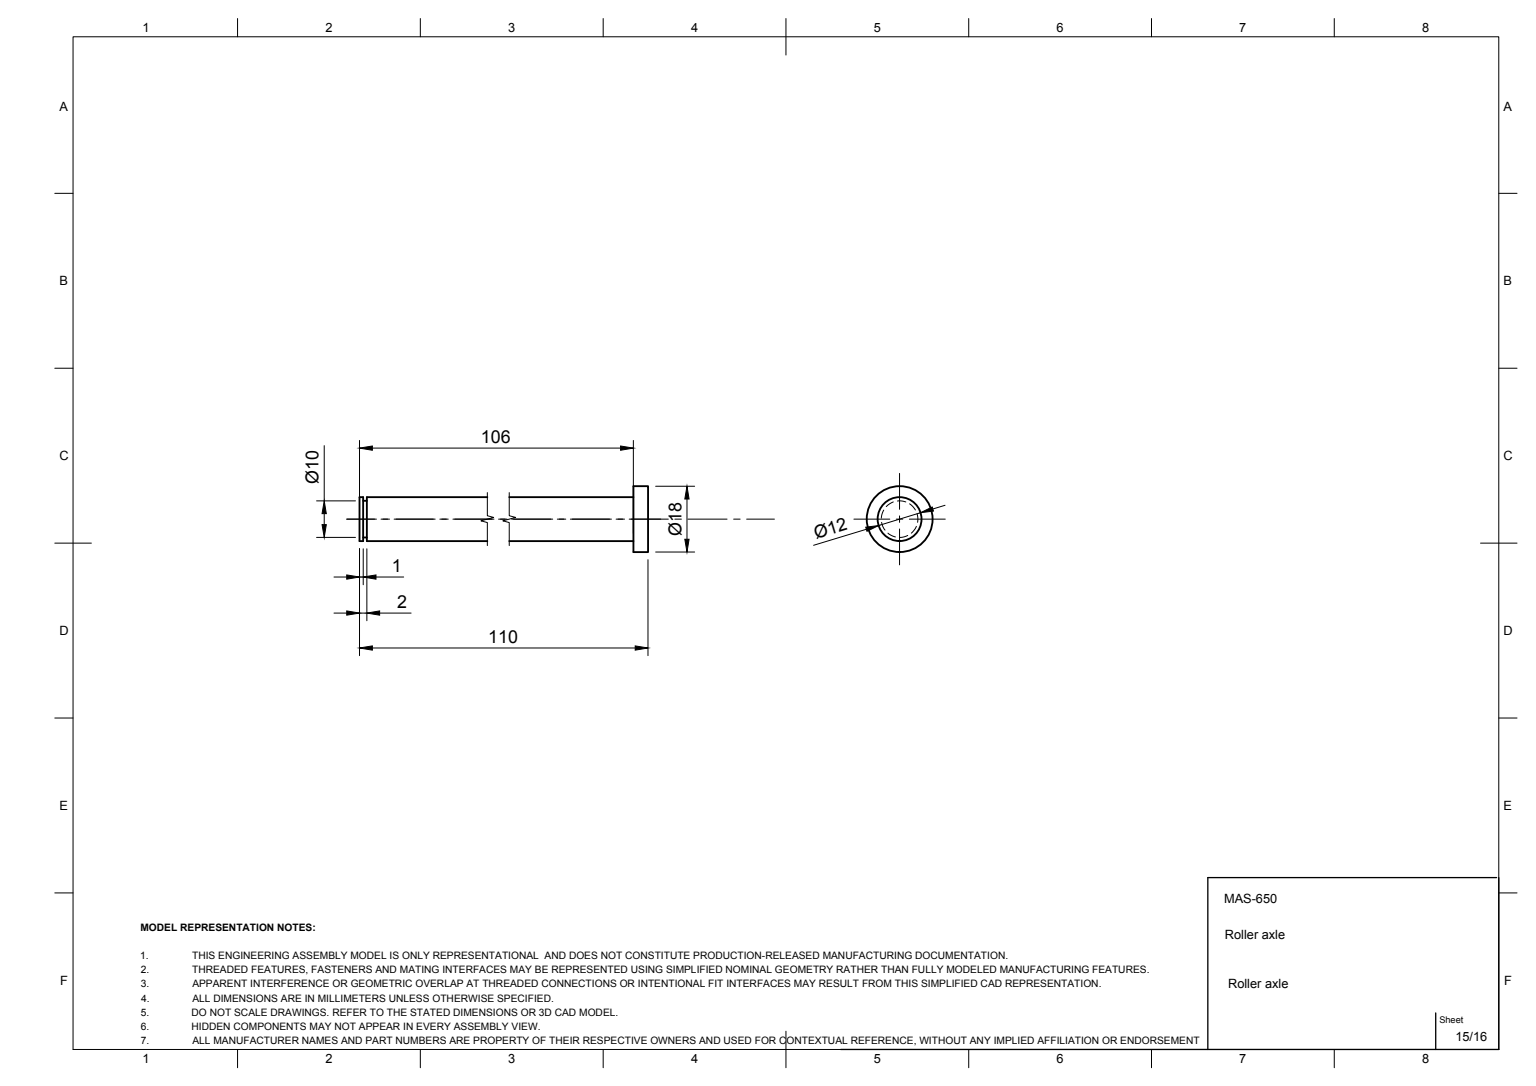
ISO-10303-21;
HEADER;
/* Generated by software containing ST-Developer
 * from STEP Tools, Inc. (www.steptools.com) 
 */

FILE_DESCRIPTION(
/* description */ ('Independent manual traversing gantry with native reusable aluminum pr
ofiles,180mm captured carriage travel, four bronze-bushed rollers, lin
ked ideal rolling motion, bonded acetal lateral guides, positive welde
d end stops and fully retained axle stacks. Editable native profile cu
t lengths220/400mm. Tool attachments viaM6 bridge-plate taps; mounted 
tool outside assembly. Welds, anchors, adhesives, fits, traction, load
/speed/structural/life ratings unassigned.'),
/* implementation_level */ '2;1');

FILE_NAME(
/* name */ 'Roller axle.step',
/* time_stamp */ '2026-11-09T20:04:38-08:00',
/* author */ (''),
/* organization */ (''),
/* preprocessor_version */ 'ST-DEVELOPER v20.2',
/* originating_system */ 'Autodesk Translation Framework v15.17.0.0',
/* authorisation */ '');

FILE_SCHEMA (('AUTOMOTIVE_DESIGN { 1 0 10303 214 3 1 1 }'));
ENDSEC;

DATA;
#10=MECHANICAL_DESIGN_GEOMETRIC_PRESENTATION_REPRESENTATION('',(#482),#13231);
#450=SHAPE_REPRESENTATION_RELATIONSHIP('SRR','None',#13339,#466);
#466=ADVANCED_BREP_SHAPE_REPRESENTATION('',(#498),#13226);
#482=STYLED_ITEM('',(#13427),#498);
#498=MANIFOLD_SOLID_BREP('Body1',#4162);
#543=FACE_BOUND('',#1090,.T.);
#544=FACE_BOUND('',#1092,.T.);
#545=FACE_BOUND('',#1095,.T.);
#618=PLANE('',#4626);
#619=PLANE('',#4628);
#620=PLANE('',#4632);
#621=PLANE('',#4637);
#622=PLANE('',#4639);
#827=FACE_OUTER_BOUND('',#1088,.T.);
#828=FACE_OUTER_BOUND('',#1089,.T.);
#829=FACE_OUTER_BOUND('',#1091,.T.);
#830=FACE_OUTER_BOUND('',#1093,.T.);
#831=FACE_OUTER_BOUND('',#1094,.T.);
#832=FACE_OUTER_BOUND('',#1096,.T.);
#833=FACE_OUTER_BOUND('',#1097,.T.);
#834=FACE_OUTER_BOUND('',#1098,.T.);
#835=FACE_OUTER_BOUND('',#1099,.T.);
#1088=EDGE_LOOP('',(#3714,#3715,#3716,#3717));
#1089=EDGE_LOOP('',(#3718));
#1090=EDGE_LOOP('',(#3719));
#1091=EDGE_LOOP('',(#3720));
#1092=EDGE_LOOP('',(#3721));
#1093=EDGE_LOOP('',(#3722,#3723,#3724,#3725));
#1094=EDGE_LOOP('',(#3726));
#1095=EDGE_LOOP('',(#3727));
#1096=EDGE_LOOP('',(#3728,#3729,#3730,#3731));
#1097=EDGE_LOOP('',(#3732));
#1098=EDGE_LOOP('',(#3733,#3734,#3735,#3736));
#1099=EDGE_LOOP('',(#3737));
#1368=LINE('',#13042,#1630);
#1369=LINE('',#13053,#1631);
#1370=LINE('',#13061,#1632);
#1371=LINE('',#13065,#1633);
#1630=VECTOR('',#5541,5.);
#1631=VECTOR('',#5556,6.);
#1632=VECTOR('',#5565,9.);
#1633=VECTOR('',#5572,6.);
#1728=CIRCLE('',#4624,5.);
#1729=CIRCLE('',#4625,5.);
#1730=CIRCLE('',#4627,6.);
#1731=CIRCLE('',#4629,6.);
#1732=CIRCLE('',#4631,6.);
#1733=CIRCLE('',#4633,9.);
#1734=CIRCLE('',#4634,6.);
#1735=CIRCLE('',#4636,9.);
#2096=VERTEX_POINT('',#13039);
#2097=VERTEX_POINT('',#13041);
#2098=VERTEX_POINT('',#13045);
#2099=VERTEX_POINT('',#13048);
#2100=VERTEX_POINT('',#13051);
#2101=VERTEX_POINT('',#13055);
#2102=VERTEX_POINT('',#13057);
#2103=VERTEX_POINT('',#13060);
#2640=EDGE_CURVE('',#2096,#2096,#1728,.T.);
#2641=EDGE_CURVE('',#2096,#2097,#1368,.T.);
#2642=EDGE_CURVE('',#2097,#2097,#1729,.T.);
#2643=EDGE_CURVE('',#2098,#2098,#1730,.T.);
#2644=EDGE_CURVE('',#2099,#2099,#1731,.T.);
#2645=EDGE_CURVE('',#2100,#2100,#1732,.T.);
#2646=EDGE_CURVE('',#2100,#2099,#1369,.T.);
#2647=EDGE_CURVE('',#2101,#2101,#1733,.T.);
#2648=EDGE_CURVE('',#2102,#2102,#1734,.T.);
#2649=EDGE_CURVE('',#2101,#2103,#1370,.T.);
#2650=EDGE_CURVE('',#2103,#2103,#1735,.T.);
#2651=EDGE_CURVE('',#2098,#2102,#1371,.T.);
#3714=ORIENTED_EDGE('',*,*,#2640,.T.);
#3715=ORIENTED_EDGE('',*,*,#2641,.T.);
#3716=ORIENTED_EDGE('',*,*,#2642,.F.);
#3717=ORIENTED_EDGE('',*,*,#2641,.F.);
#3718=ORIENTED_EDGE('',*,*,#2643,.F.);
#3719=ORIENTED_EDGE('',*,*,#2640,.F.);
#3720=ORIENTED_EDGE('',*,*,#2644,.F.);
#3721=ORIENTED_EDGE('',*,*,#2642,.T.);
#3722=ORIENTED_EDGE('',*,*,#2645,.F.);
#3723=ORIENTED_EDGE('',*,*,#2646,.T.);
#3724=ORIENTED_EDGE('',*,*,#2644,.T.);
#3725=ORIENTED_EDGE('',*,*,#2646,.F.);
#3726=ORIENTED_EDGE('',*,*,#2647,.T.);
#3727=ORIENTED_EDGE('',*,*,#2648,.F.);
#3728=ORIENTED_EDGE('',*,*,#2647,.F.);
#3729=ORIENTED_EDGE('',*,*,#2649,.T.);
#3730=ORIENTED_EDGE('',*,*,#2650,.T.);
#3731=ORIENTED_EDGE('',*,*,#2649,.F.);
#3732=ORIENTED_EDGE('',*,*,#2650,.F.);
#3733=ORIENTED_EDGE('',*,*,#2643,.T.);
#3734=ORIENTED_EDGE('',*,*,#2651,.T.);
#3735=ORIENTED_EDGE('',*,*,#2648,.T.);
#3736=ORIENTED_EDGE('',*,*,#2651,.F.);
#3737=ORIENTED_EDGE('',*,*,#2645,.T.);
#3918=CYLINDRICAL_SURFACE('',#4623,5.);
#3919=CYLINDRICAL_SURFACE('',#4630,6.);
#3920=CYLINDRICAL_SURFACE('',#4635,9.);
#3921=CYLINDRICAL_SURFACE('',#4638,6.);
#4124=ADVANCED_FACE('',(#827),#3918,.T.);
#4125=ADVANCED_FACE('',(#828,#543),#618,.F.);
#4126=ADVANCED_FACE('',(#829,#544),#619,.F.);
#4127=ADVANCED_FACE('',(#830),#3919,.T.);
#4128=ADVANCED_FACE('',(#831,#545),#620,.T.);
#4129=ADVANCED_FACE('',(#832),#3920,.T.);
#4130=ADVANCED_FACE('',(#833),#621,.F.);
#4131=ADVANCED_FACE('',(#834),#3921,.T.);
#4132=ADVANCED_FACE('',(#835),#622,.T.);
#4162=CLOSED_SHELL('',(#4124,#4125,#4126,#4127,#4128,#4129,#4130,#4131,
#4132));
#4622=AXIS2_PLACEMENT_3D('',#13037,#5535,#5536);
#4623=AXIS2_PLACEMENT_3D('',#13038,#5537,#5538);
#4624=AXIS2_PLACEMENT_3D('',#13040,#5539,#5540);
#4625=AXIS2_PLACEMENT_3D('',#13043,#5542,#5543);
#4626=AXIS2_PLACEMENT_3D('',#13044,#5544,#5545);
#4627=AXIS2_PLACEMENT_3D('',#13046,#5546,#5547);
#4628=AXIS2_PLACEMENT_3D('',#13047,#5548,#5549);
#4629=AXIS2_PLACEMENT_3D('',#13049,#5550,#5551);
#4630=AXIS2_PLACEMENT_3D('',#13050,#5552,#5553);
#4631=AXIS2_PLACEMENT_3D('',#13052,#5554,#5555);
#4632=AXIS2_PLACEMENT_3D('',#13054,#5557,#5558);
#4633=AXIS2_PLACEMENT_3D('',#13056,#5559,#5560);
#4634=AXIS2_PLACEMENT_3D('',#13058,#5561,#5562);
#4635=AXIS2_PLACEMENT_3D('',#13059,#5563,#5564);
#4636=AXIS2_PLACEMENT_3D('',#13062,#5566,#5567);
#4637=AXIS2_PLACEMENT_3D('',#13063,#5568,#5569);
#4638=AXIS2_PLACEMENT_3D('',#13064,#5570,#5571);
#4639=AXIS2_PLACEMENT_3D('',#13066,#5573,#5574);
#5535=DIRECTION('axis',(0.,0.,1.));
#5536=DIRECTION('refdir',(1.,0.,0.));
#5537=DIRECTION('center_axis',(0.,0.,1.));
#5538=DIRECTION('ref_axis',(1.,0.,0.));
#5539=DIRECTION('center_axis',(0.,0.,1.));
#5540=DIRECTION('ref_axis',(1.,0.,0.));
#5541=DIRECTION('',(0.,0.,1.));
#5542=DIRECTION('center_axis',(0.,0.,1.));
#5543=DIRECTION('ref_axis',(1.,0.,0.));
#5544=DIRECTION('center_axis',(0.,0.,-1.));
#5545=DIRECTION('ref_axis',(-1.,0.,0.));
#5546=DIRECTION('center_axis',(0.,0.,-1.));
#5547=DIRECTION('ref_axis',(1.,0.,0.));
#5548=DIRECTION('center_axis',(0.,0.,1.));
#5549=DIRECTION('ref_axis',(1.,0.,0.));
#5550=DIRECTION('center_axis',(0.,0.,1.));
#5551=DIRECTION('ref_axis',(1.,0.,0.));
#5552=DIRECTION('center_axis',(0.,0.,1.));
#5553=DIRECTION('ref_axis',(1.,0.,0.));
#5554=DIRECTION('center_axis',(0.,0.,1.));
#5555=DIRECTION('ref_axis',(1.,0.,0.));
#5556=DIRECTION('',(0.,0.,-1.));
#5557=DIRECTION('center_axis',(0.,0.,1.));
#5558=DIRECTION('ref_axis',(1.,0.,0.));
#5559=DIRECTION('center_axis',(0.,0.,1.));
#5560=DIRECTION('ref_axis',(1.,0.,0.));
#5561=DIRECTION('center_axis',(0.,0.,1.));
#5562=DIRECTION('ref_axis',(1.,0.,0.));
#5563=DIRECTION('center_axis',(0.,0.,1.));
#5564=DIRECTION('ref_axis',(1.,0.,0.));
#5565=DIRECTION('',(0.,0.,-1.));
#5566=DIRECTION('center_axis',(0.,0.,1.));
#5567=DIRECTION('ref_axis',(1.,0.,0.));
#5568=DIRECTION('center_axis',(0.,0.,1.));
#5569=DIRECTION('ref_axis',(1.,0.,0.));
#5570=DIRECTION('center_axis',(0.,0.,1.));
#5571=DIRECTION('ref_axis',(1.,0.,0.));
#5572=DIRECTION('',(0.,0.,-1.));
#5573=DIRECTION('center_axis',(0.,0.,1.));
#5574=DIRECTION('ref_axis',(1.,0.,0.));
#13037=CARTESIAN_POINT('',(0.,0.,0.));
#13038=CARTESIAN_POINT('Origin',(0.,0.,104.5));
#13039=CARTESIAN_POINT('',(-5.,-6.12323399573677E-16,104.));
#13040=CARTESIAN_POINT('Origin',(0.,0.,104.));
#13041=CARTESIAN_POINT('',(-5.,-6.12323399573677E-16,105.));
#13042=CARTESIAN_POINT('',(-5.,-6.12323399573677E-16,104.5));
#13043=CARTESIAN_POINT('Origin',(0.,0.,105.));
#13044=CARTESIAN_POINT('Origin',(9.,0.,104.));
#13045=CARTESIAN_POINT('',(-6.,7.34788079488412E-16,104.));
#13046=CARTESIAN_POINT('Origin',(0.,0.,104.));
#13047=CARTESIAN_POINT('Origin',(5.,0.,105.));
#13048=CARTESIAN_POINT('',(-6.,-7.34788079488412E-16,105.));
#13049=CARTESIAN_POINT('Origin',(0.,0.,105.));
#13050=CARTESIAN_POINT('Origin',(0.,0.,0.));
#13051=CARTESIAN_POINT('',(-6.,-7.34788079488412E-16,106.));
#13052=CARTESIAN_POINT('Origin',(0.,0.,106.));
#13053=CARTESIAN_POINT('',(-6.,-7.34788079488412E-16,0.));
#13054=CARTESIAN_POINT('Origin',(0.,0.,0.));
#13055=CARTESIAN_POINT('',(-9.,-1.10218211923262E-15,0.));
#13056=CARTESIAN_POINT('Origin',(0.,0.,0.));
#13057=CARTESIAN_POINT('',(-6.,-7.34788079488412E-16,0.));
#13058=CARTESIAN_POINT('Origin',(0.,0.,0.));
#13059=CARTESIAN_POINT('Origin',(0.,0.,-4.));
#13060=CARTESIAN_POINT('',(-9.,-1.10218211923262E-15,-4.));
#13061=CARTESIAN_POINT('',(-9.,-1.10218211923262E-15,-4.));
#13062=CARTESIAN_POINT('Origin',(0.,0.,-4.));
#13063=CARTESIAN_POINT('Origin',(0.,0.,-4.));
#13064=CARTESIAN_POINT('Origin',(0.,0.,0.));
#13065=CARTESIAN_POINT('',(-6.,-7.34788079488412E-16,0.));
#13066=CARTESIAN_POINT('Origin',(0.,0.,106.));
#13208=UNCERTAINTY_MEASURE_WITH_UNIT(LENGTH_MEASURE(0.01),#13232,
'DISTANCE_ACCURACY_VALUE',
'Maximum model space distance between geometric entities at asserted c
onnectivities');
#13213=UNCERTAINTY_MEASURE_WITH_UNIT(LENGTH_MEASURE(0.01),#13232,
'DISTANCE_ACCURACY_VALUE',
'Maximum model space distance between geometric entities at asserted c
onnectivities');
#13226=(
GEOMETRIC_REPRESENTATION_CONTEXT(3)
GLOBAL_UNCERTAINTY_ASSIGNED_CONTEXT((#13208))
GLOBAL_UNIT_ASSIGNED_CONTEXT((#13232,#13234,#13235))
REPRESENTATION_CONTEXT('','3D')
);
#13231=(
GEOMETRIC_REPRESENTATION_CONTEXT(3)
GLOBAL_UNCERTAINTY_ASSIGNED_CONTEXT((#13213))
GLOBAL_UNIT_ASSIGNED_CONTEXT((#13232,#13234,#13235))
REPRESENTATION_CONTEXT('','3D')
);
#13232=(
LENGTH_UNIT()
NAMED_UNIT(*)
SI_UNIT(.MILLI.,.METRE.)
);
#13234=(
NAMED_UNIT(*)
PLANE_ANGLE_UNIT()
SI_UNIT($,.RADIAN.)
);
#13235=(
NAMED_UNIT(*)
SI_UNIT($,.STERADIAN.)
SOLID_ANGLE_UNIT()
);
#13248=SHAPE_DEFINITION_REPRESENTATION(#13265,#13339);
#13265=PRODUCT_DEFINITION_SHAPE('',$,#13357);
#13339=SHAPE_REPRESENTATION('',(#4622),#13226);
#13344=PRODUCT_DEFINITION_CONTEXT('part definition',#13397,'design');
#13357=PRODUCT_DEFINITION('Roller axle','Roller axle',#13374,#13344);
#13374=PRODUCT_DEFINITION_FORMATION('',$,#13411);
#13397=APPLICATION_CONTEXT(
'Core Data for Automotive Mechanical Design Process');
#13398=PRODUCT_CONTEXT('part definition',#13397,'mechanical');
#13411=PRODUCT('Roller axle','Roller axle','Roller axle',(#13398));
#13427=PRESENTATION_STYLE_ASSIGNMENT((#13441));
#13441=SURFACE_STYLE_USAGE(.BOTH.,#13455);
#13455=SURFACE_SIDE_STYLE('',(#13469));
#13469=SURFACE_STYLE_FILL_AREA(#13483);
#13483=FILL_AREA_STYLE('Axle gray',(#13497));
#13497=FILL_AREA_STYLE_COLOUR('Axle gray',#13511);
#13511=COLOUR_RGB('Axle gray',0.576470588235294,0.615686274509804,0.666666666666667);
ENDSEC;
END-ISO-10303-21;
